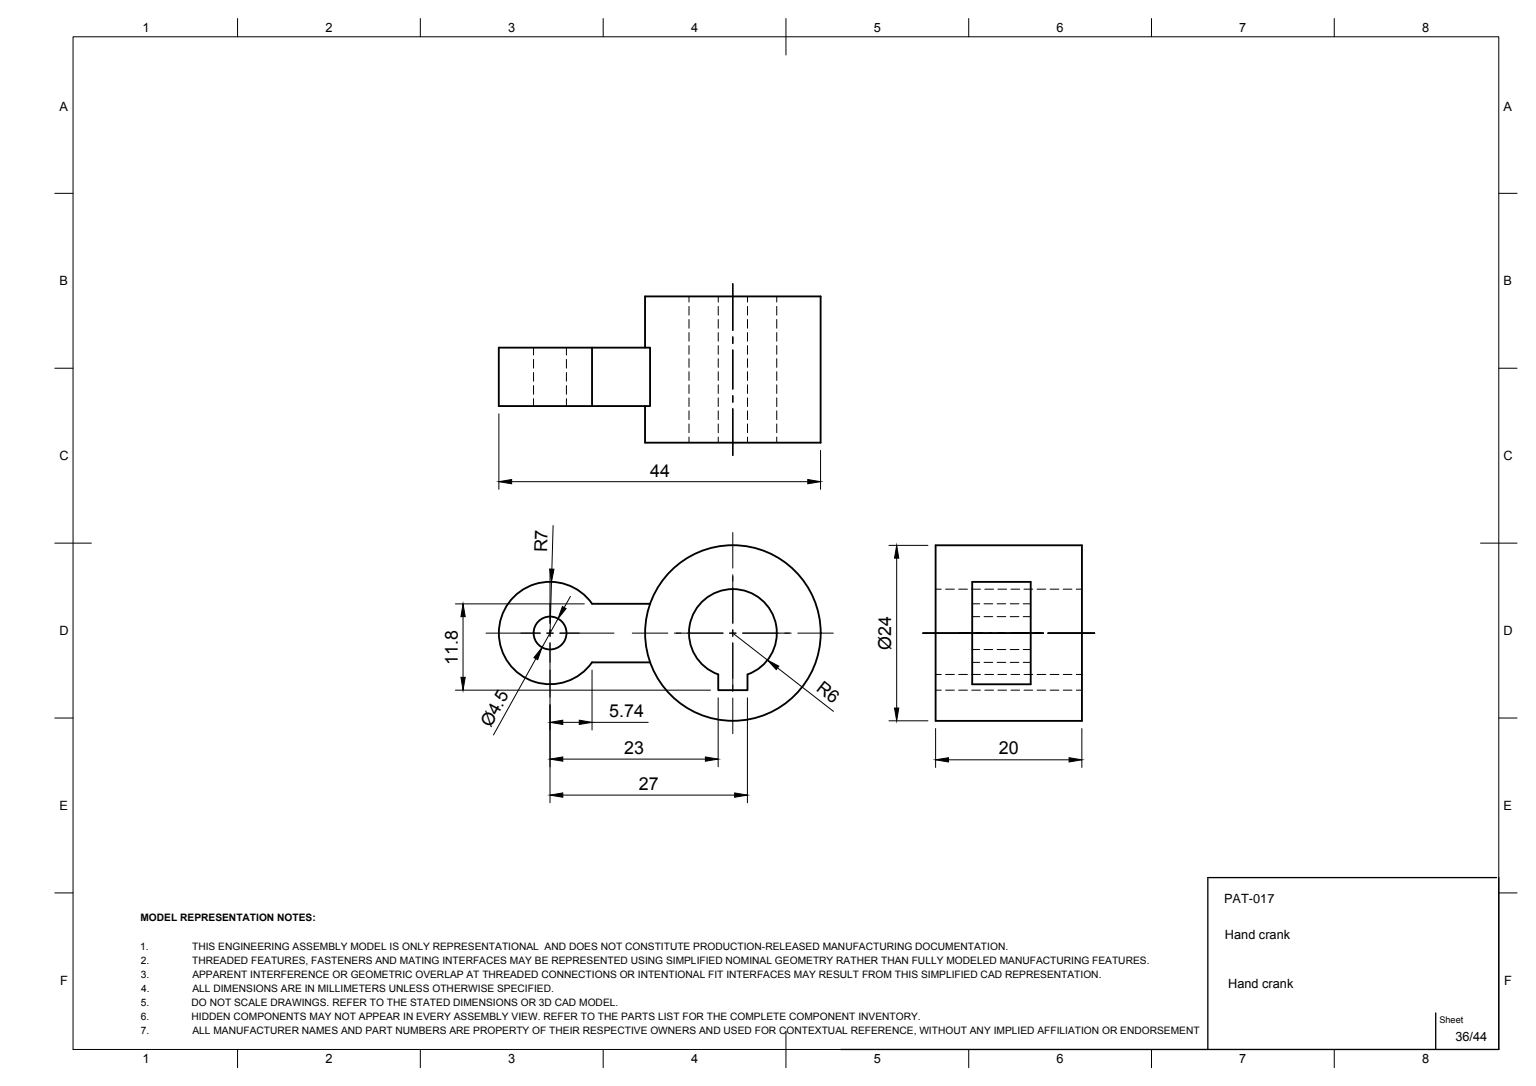
ISO-10303-21;
HEADER;
/* Generated by software containing ST-Developer
 * from STEP Tools, Inc. (www.steptools.com) 
 */

FILE_DESCRIPTION(
/* description */ ('Cam-and-follower valve demonstrator'),
/* implementation_level */ '2;1');

FILE_NAME(
/* name */ 'Hand crank.step',
/* time_stamp */ '2026-10-28T03:25:17-07:00',
/* author */ (''),
/* organization */ (''),
/* preprocessor_version */ 'ST-DEVELOPER v20.2',
/* originating_system */ 'Autodesk Translation Framework v15.17.0.0',
/* authorisation */ '');

FILE_SCHEMA (('AUTOMOTIVE_DESIGN { 1 0 10303 214 3 1 1 }'));
ENDSEC;

DATA;
#10=MECHANICAL_DESIGN_GEOMETRIC_PRESENTATION_REPRESENTATION('',(#446),#12896);
#367=SHAPE_REPRESENTATION_RELATIONSHIP('SRR','None',#13086,#403);
#403=ADVANCED_BREP_SHAPE_REPRESENTATION('',(#487),#12886);
#446=STYLED_ITEM('',(#13316),#487);
#487=MANIFOLD_SOLID_BREP('Body1',#6215);
#642=FACE_BOUND('',#1912,.T.);
#643=FACE_BOUND('',#1916,.T.);
#644=FACE_BOUND('',#1920,.T.);
#645=FACE_BOUND('',#1922,.T.);
#646=FACE_BOUND('',#1924,.T.);
#931=CIRCLE('',#7231,0.225);
#932=CIRCLE('',#7232,0.225);
#933=CIRCLE('',#7237,1.2);
#934=CIRCLE('',#7238,0.6);
#935=CIRCLE('',#7240,0.6);
#936=CIRCLE('',#7242,0.7);
#937=CIRCLE('',#7243,0.7);
#938=CIRCLE('',#7245,1.2);
#939=CIRCLE('',#7249,1.2);
#940=CIRCLE('',#7251,1.2);
#1077=CYLINDRICAL_SURFACE('',#7230,0.225);
#1078=CYLINDRICAL_SURFACE('',#7239,0.6);
#1079=CYLINDRICAL_SURFACE('',#7241,0.7);
#1080=CYLINDRICAL_SURFACE('',#7250,1.2);
#1392=FACE_OUTER_BOUND('',#1907,.T.);
#1393=FACE_OUTER_BOUND('',#1908,.T.);
#1394=FACE_OUTER_BOUND('',#1909,.T.);
#1395=FACE_OUTER_BOUND('',#1910,.T.);
#1396=FACE_OUTER_BOUND('',#1911,.T.);
#1397=FACE_OUTER_BOUND('',#1913,.T.);
#1398=FACE_OUTER_BOUND('',#1914,.T.);
#1399=FACE_OUTER_BOUND('',#1915,.T.);
#1400=FACE_OUTER_BOUND('',#1917,.T.);
#1401=FACE_OUTER_BOUND('',#1918,.T.);
#1402=FACE_OUTER_BOUND('',#1919,.T.);
#1403=FACE_OUTER_BOUND('',#1921,.T.);
#1404=FACE_OUTER_BOUND('',#1923,.T.);
#1907=EDGE_LOOP('',(#5329,#5330,#5331,#5332));
#1908=EDGE_LOOP('',(#5333,#5334,#5335,#5336));
#1909=EDGE_LOOP('',(#5337,#5338,#5339,#5340));
#1910=EDGE_LOOP('',(#5341,#5342,#5343,#5344));
#1911=EDGE_LOOP('',(#5345));
#1912=EDGE_LOOP('',(#5346,#5347,#5348,#5349));
#1913=EDGE_LOOP('',(#5350,#5351,#5352,#5353));
#1914=EDGE_LOOP('',(#5354,#5355,#5356,#5357));
#1915=EDGE_LOOP('',(#5358,#5359,#5360,#5361));
#1916=EDGE_LOOP('',(#5362));
#1917=EDGE_LOOP('',(#5363,#5364,#5365,#5366));
#1918=EDGE_LOOP('',(#5367,#5368,#5369,#5370));
#1919=EDGE_LOOP('',(#5371,#5372,#5373,#5374));
#1920=EDGE_LOOP('',(#5375));
#1921=EDGE_LOOP('',(#5376,#5377,#5378,#5379));
#1922=EDGE_LOOP('',(#5380,#5381,#5382,#5383));
#1923=EDGE_LOOP('',(#5384));
#1924=EDGE_LOOP('',(#5385,#5386,#5387,#5388));
#2325=LINE('',#12451,#2747);
#2326=LINE('',#12456,#2748);
#2327=LINE('',#12458,#2749);
#2328=LINE('',#12460,#2750);
#2329=LINE('',#12461,#2751);
#2330=LINE('',#12464,#2752);
#2331=LINE('',#12466,#2753);
#2332=LINE('',#12467,#2754);
#2333=LINE('',#12470,#2755);
#2334=LINE('',#12472,#2756);
#2335=LINE('',#12473,#2757);
#2336=LINE('',#12483,#2758);
#2337=LINE('',#12487,#2759);
#2338=LINE('',#12491,#2760);
#2339=LINE('',#12494,#2761);
#2340=LINE('',#12497,#2762);
#2341=LINE('',#12498,#2763);
#2342=LINE('',#12501,#2764);
#2343=LINE('',#12502,#2765);
#2344=LINE('',#12507,#2766);
#2747=VECTOR('',#8964,0.225);
#2748=VECTOR('',#8969,1.);
#2749=VECTOR('',#8970,1.);
#2750=VECTOR('',#8971,1.);
#2751=VECTOR('',#8972,1.);
#2752=VECTOR('',#8975,1.);
#2753=VECTOR('',#8976,1.);
#2754=VECTOR('',#8977,1.);
#2755=VECTOR('',#8980,1.);
#2756=VECTOR('',#8981,1.);
#2757=VECTOR('',#8982,1.);
#2758=VECTOR('',#8995,1.);
#2759=VECTOR('',#8998,1.);
#2760=VECTOR('',#9003,1.);
#2761=VECTOR('',#9006,1.);
#2762=VECTOR('',#9009,1.);
#2763=VECTOR('',#9010,1.);
#2764=VECTOR('',#9013,1.);
#2765=VECTOR('',#9014,1.);
#2766=VECTOR('',#9021,1.2);
#3256=VERTEX_POINT('',#12448);
#3257=VERTEX_POINT('',#12450);
#3258=VERTEX_POINT('',#12454);
#3259=VERTEX_POINT('',#12455);
#3260=VERTEX_POINT('',#12457);
#3261=VERTEX_POINT('',#12459);
#3262=VERTEX_POINT('',#12463);
#3263=VERTEX_POINT('',#12465);
#3264=VERTEX_POINT('',#12469);
#3265=VERTEX_POINT('',#12471);
#3266=VERTEX_POINT('',#12475);
#3267=VERTEX_POINT('',#12481);
#3268=VERTEX_POINT('',#12482);
#3269=VERTEX_POINT('',#12484);
#3270=VERTEX_POINT('',#12486);
#3271=VERTEX_POINT('',#12490);
#3272=VERTEX_POINT('',#12492);
#3273=VERTEX_POINT('',#12496);
#3274=VERTEX_POINT('',#12500);
#3275=VERTEX_POINT('',#12506);
#3961=EDGE_CURVE('',#3256,#3256,#931,.T.);
#3962=EDGE_CURVE('',#3256,#3257,#2325,.T.);
#3963=EDGE_CURVE('',#3257,#3257,#932,.T.);
#3964=EDGE_CURVE('',#3258,#3259,#2326,.T.);
#3965=EDGE_CURVE('',#3258,#3260,#2327,.T.);
#3966=EDGE_CURVE('',#3261,#3260,#2328,.T.);
#3967=EDGE_CURVE('',#3259,#3261,#2329,.T.);
#3968=EDGE_CURVE('',#3262,#3258,#2330,.T.);
#3969=EDGE_CURVE('',#3262,#3263,#2331,.T.);
#3970=EDGE_CURVE('',#3260,#3263,#2332,.T.);
#3971=EDGE_CURVE('',#3264,#3262,#2333,.T.);
#3972=EDGE_CURVE('',#3265,#3264,#2334,.T.);
#3973=EDGE_CURVE('',#3263,#3265,#2335,.T.);
#3974=EDGE_CURVE('',#3266,#3266,#933,.T.);
#3975=EDGE_CURVE('',#3265,#3261,#934,.T.);
#3976=EDGE_CURVE('',#3264,#3259,#935,.T.);
#3977=EDGE_CURVE('',#3267,#3268,#2336,.T.);
#3978=EDGE_CURVE('',#3269,#3267,#936,.T.);
#3979=EDGE_CURVE('',#3270,#3269,#2337,.T.);
#3980=EDGE_CURVE('',#3270,#3268,#937,.T.);
#3981=EDGE_CURVE('',#3270,#3271,#2338,.T.);
#3982=EDGE_CURVE('',#3272,#3271,#938,.T.);
#3983=EDGE_CURVE('',#3272,#3268,#2339,.T.);
#3984=EDGE_CURVE('',#3273,#3269,#2340,.T.);
#3985=EDGE_CURVE('',#3271,#3273,#2341,.T.);
#3986=EDGE_CURVE('',#3274,#3272,#2342,.T.);
#3987=EDGE_CURVE('',#3267,#3274,#2343,.T.);
#3988=EDGE_CURVE('',#3273,#3274,#939,.T.);
#3989=EDGE_CURVE('',#3266,#3275,#2344,.T.);
#3990=EDGE_CURVE('',#3275,#3275,#940,.T.);
#5329=ORIENTED_EDGE('',*,*,#3961,.F.);
#5330=ORIENTED_EDGE('',*,*,#3962,.T.);
#5331=ORIENTED_EDGE('',*,*,#3963,.F.);
#5332=ORIENTED_EDGE('',*,*,#3962,.F.);
#5333=ORIENTED_EDGE('',*,*,#3964,.F.);
#5334=ORIENTED_EDGE('',*,*,#3965,.T.);
#5335=ORIENTED_EDGE('',*,*,#3966,.F.);
#5336=ORIENTED_EDGE('',*,*,#3967,.F.);
#5337=ORIENTED_EDGE('',*,*,#3968,.F.);
#5338=ORIENTED_EDGE('',*,*,#3969,.T.);
#5339=ORIENTED_EDGE('',*,*,#3970,.F.);
#5340=ORIENTED_EDGE('',*,*,#3965,.F.);
#5341=ORIENTED_EDGE('',*,*,#3971,.F.);
#5342=ORIENTED_EDGE('',*,*,#3972,.F.);
#5343=ORIENTED_EDGE('',*,*,#3973,.F.);
#5344=ORIENTED_EDGE('',*,*,#3969,.F.);
#5345=ORIENTED_EDGE('',*,*,#3974,.T.);
#5346=ORIENTED_EDGE('',*,*,#3966,.T.);
#5347=ORIENTED_EDGE('',*,*,#3970,.T.);
#5348=ORIENTED_EDGE('',*,*,#3973,.T.);
#5349=ORIENTED_EDGE('',*,*,#3975,.T.);
#5350=ORIENTED_EDGE('',*,*,#3967,.T.);
#5351=ORIENTED_EDGE('',*,*,#3975,.F.);
#5352=ORIENTED_EDGE('',*,*,#3972,.T.);
#5353=ORIENTED_EDGE('',*,*,#3976,.T.);
#5354=ORIENTED_EDGE('',*,*,#3977,.F.);
#5355=ORIENTED_EDGE('',*,*,#3978,.F.);
#5356=ORIENTED_EDGE('',*,*,#3979,.F.);
#5357=ORIENTED_EDGE('',*,*,#3980,.T.);
#5358=ORIENTED_EDGE('',*,*,#3980,.F.);
#5359=ORIENTED_EDGE('',*,*,#3981,.T.);
#5360=ORIENTED_EDGE('',*,*,#3982,.F.);
#5361=ORIENTED_EDGE('',*,*,#3983,.T.);
#5362=ORIENTED_EDGE('',*,*,#3961,.T.);
#5363=ORIENTED_EDGE('',*,*,#3979,.T.);
#5364=ORIENTED_EDGE('',*,*,#3984,.F.);
#5365=ORIENTED_EDGE('',*,*,#3985,.F.);
#5366=ORIENTED_EDGE('',*,*,#3981,.F.);
#5367=ORIENTED_EDGE('',*,*,#3977,.T.);
#5368=ORIENTED_EDGE('',*,*,#3983,.F.);
#5369=ORIENTED_EDGE('',*,*,#3986,.F.);
#5370=ORIENTED_EDGE('',*,*,#3987,.F.);
#5371=ORIENTED_EDGE('',*,*,#3987,.T.);
#5372=ORIENTED_EDGE('',*,*,#3988,.F.);
#5373=ORIENTED_EDGE('',*,*,#3984,.T.);
#5374=ORIENTED_EDGE('',*,*,#3978,.T.);
#5375=ORIENTED_EDGE('',*,*,#3963,.T.);
#5376=ORIENTED_EDGE('',*,*,#3974,.F.);
#5377=ORIENTED_EDGE('',*,*,#3989,.T.);
#5378=ORIENTED_EDGE('',*,*,#3990,.T.);
#5379=ORIENTED_EDGE('',*,*,#3989,.F.);
#5380=ORIENTED_EDGE('',*,*,#3985,.T.);
#5381=ORIENTED_EDGE('',*,*,#3988,.T.);
#5382=ORIENTED_EDGE('',*,*,#3986,.T.);
#5383=ORIENTED_EDGE('',*,*,#3982,.T.);
#5384=ORIENTED_EDGE('',*,*,#3990,.F.);
#5385=ORIENTED_EDGE('',*,*,#3964,.T.);
#5386=ORIENTED_EDGE('',*,*,#3976,.F.);
#5387=ORIENTED_EDGE('',*,*,#3971,.T.);
#5388=ORIENTED_EDGE('',*,*,#3968,.T.);
#5762=PLANE('',#7233);
#5763=PLANE('',#7234);
#5764=PLANE('',#7235);
#5765=PLANE('',#7236);
#5766=PLANE('',#7244);
#5767=PLANE('',#7246);
#5768=PLANE('',#7247);
#5769=PLANE('',#7248);
#5770=PLANE('',#7252);
#6108=ADVANCED_FACE('',(#1392),#1077,.F.);
#6109=ADVANCED_FACE('',(#1393),#5762,.F.);
#6110=ADVANCED_FACE('',(#1394),#5763,.F.);
#6111=ADVANCED_FACE('',(#1395),#5764,.F.);
#6112=ADVANCED_FACE('',(#1396,#642),#5765,.T.);
#6113=ADVANCED_FACE('',(#1397),#1078,.F.);
#6114=ADVANCED_FACE('',(#1398),#1079,.T.);
#6115=ADVANCED_FACE('',(#1399,#643),#5766,.F.);
#6116=ADVANCED_FACE('',(#1400),#5767,.T.);
#6117=ADVANCED_FACE('',(#1401),#5768,.T.);
#6118=ADVANCED_FACE('',(#1402,#644),#5769,.T.);
#6119=ADVANCED_FACE('',(#1403,#645),#1080,.T.);
#6120=ADVANCED_FACE('',(#1404,#646),#5770,.F.);
#6215=CLOSED_SHELL('',(#6108,#6109,#6110,#6111,#6112,#6113,#6114,#6115,
#6116,#6117,#6118,#6119,#6120));
#7229=AXIS2_PLACEMENT_3D('',#12446,#8958,#8959);
#7230=AXIS2_PLACEMENT_3D('',#12447,#8960,#8961);
#7231=AXIS2_PLACEMENT_3D('',#12449,#8962,#8963);
#7232=AXIS2_PLACEMENT_3D('',#12452,#8965,#8966);
#7233=AXIS2_PLACEMENT_3D('',#12453,#8967,#8968);
#7234=AXIS2_PLACEMENT_3D('',#12462,#8973,#8974);
#7235=AXIS2_PLACEMENT_3D('',#12468,#8978,#8979);
#7236=AXIS2_PLACEMENT_3D('',#12474,#8983,#8984);
#7237=AXIS2_PLACEMENT_3D('',#12476,#8985,#8986);
#7238=AXIS2_PLACEMENT_3D('',#12477,#8987,#8988);
#7239=AXIS2_PLACEMENT_3D('',#12478,#8989,#8990);
#7240=AXIS2_PLACEMENT_3D('',#12479,#8991,#8992);
#7241=AXIS2_PLACEMENT_3D('',#12480,#8993,#8994);
#7242=AXIS2_PLACEMENT_3D('',#12485,#8996,#8997);
#7243=AXIS2_PLACEMENT_3D('',#12488,#8999,#9000);
#7244=AXIS2_PLACEMENT_3D('',#12489,#9001,#9002);
#7245=AXIS2_PLACEMENT_3D('',#12493,#9004,#9005);
#7246=AXIS2_PLACEMENT_3D('',#12495,#9007,#9008);
#7247=AXIS2_PLACEMENT_3D('',#12499,#9011,#9012);
#7248=AXIS2_PLACEMENT_3D('',#12503,#9015,#9016);
#7249=AXIS2_PLACEMENT_3D('',#12504,#9017,#9018);
#7250=AXIS2_PLACEMENT_3D('',#12505,#9019,#9020);
#7251=AXIS2_PLACEMENT_3D('',#12508,#9022,#9023);
#7252=AXIS2_PLACEMENT_3D('',#12509,#9024,#9025);
#8958=DIRECTION('axis',(0.,0.,1.));
#8959=DIRECTION('refdir',(1.,0.,0.));
#8960=DIRECTION('center_axis',(0.,1.,0.));
#8961=DIRECTION('ref_axis',(1.,0.,0.));
#8962=DIRECTION('center_axis',(0.,1.,0.));
#8963=DIRECTION('ref_axis',(1.,0.,0.));
#8964=DIRECTION('',(0.,1.,0.));
#8965=DIRECTION('center_axis',(0.,-1.,0.));
#8966=DIRECTION('ref_axis',(1.,0.,0.));
#8967=DIRECTION('center_axis',(-1.,0.,0.));
#8968=DIRECTION('ref_axis',(0.,0.,1.));
#8969=DIRECTION('',(0.,0.,1.));
#8970=DIRECTION('',(0.,1.,0.));
#8971=DIRECTION('',(0.,0.,-1.));
#8972=DIRECTION('',(0.,1.,0.));
#8973=DIRECTION('center_axis',(0.,0.,-1.));
#8974=DIRECTION('ref_axis',(-1.,0.,0.));
#8975=DIRECTION('',(-1.,0.,0.));
#8976=DIRECTION('',(0.,1.,0.));
#8977=DIRECTION('',(1.,0.,0.));
#8978=DIRECTION('center_axis',(1.,0.,0.));
#8979=DIRECTION('ref_axis',(0.,0.,-1.));
#8980=DIRECTION('',(0.,0.,-1.));
#8981=DIRECTION('',(0.,-1.,0.));
#8982=DIRECTION('',(0.,0.,1.));
#8983=DIRECTION('center_axis',(0.,1.,0.));
#8984=DIRECTION('ref_axis',(1.,0.,0.));
#8985=DIRECTION('center_axis',(0.,1.,0.));
#8986=DIRECTION('ref_axis',(1.,0.,0.));
#8987=DIRECTION('center_axis',(0.,-1.,0.));
#8988=DIRECTION('ref_axis',(1.,0.,0.));
#8989=DIRECTION('center_axis',(0.,1.,0.));
#8990=DIRECTION('ref_axis',(-1.83697019872103E-16,0.,1.));
#8991=DIRECTION('center_axis',(0.,-1.,0.));
#8992=DIRECTION('ref_axis',(1.,0.,0.));
#8993=DIRECTION('center_axis',(0.,1.,0.));
#8994=DIRECTION('ref_axis',(1.,0.,0.));
#8995=DIRECTION('',(0.,-1.,0.));
#8996=DIRECTION('center_axis',(0.,1.,0.));
#8997=DIRECTION('ref_axis',(1.,0.,0.));
#8998=DIRECTION('',(0.,1.,0.));
#8999=DIRECTION('center_axis',(0.,1.,0.));
#9000=DIRECTION('ref_axis',(1.,0.,0.));
#9001=DIRECTION('center_axis',(0.,1.,0.));
#9002=DIRECTION('ref_axis',(1.,0.,0.));
#9003=DIRECTION('',(-1.,0.,0.));
#9004=DIRECTION('center_axis',(0.,-1.,0.));
#9005=DIRECTION('ref_axis',(1.,0.,0.));
#9006=DIRECTION('',(1.,0.,0.));
#9007=DIRECTION('center_axis',(0.,0.,1.));
#9008=DIRECTION('ref_axis',(1.,0.,0.));
#9009=DIRECTION('',(1.,0.,0.));
#9010=DIRECTION('',(0.,1.,0.));
#9011=DIRECTION('center_axis',(0.,0.,-1.));
#9012=DIRECTION('ref_axis',(-1.,0.,0.));
#9013=DIRECTION('',(0.,-1.,0.));
#9014=DIRECTION('',(-1.,0.,0.));
#9015=DIRECTION('center_axis',(0.,1.,0.));
#9016=DIRECTION('ref_axis',(0.,0.,1.));
#9017=DIRECTION('center_axis',(0.,1.,0.));
#9018=DIRECTION('ref_axis',(1.,0.,0.));
#9019=DIRECTION('center_axis',(0.,1.,0.));
#9020=DIRECTION('ref_axis',(1.,0.,0.));
#9021=DIRECTION('',(0.,-1.,0.));
#9022=DIRECTION('center_axis',(0.,1.,0.));
#9023=DIRECTION('ref_axis',(1.,0.,0.));
#9024=DIRECTION('center_axis',(0.,1.,0.));
#9025=DIRECTION('ref_axis',(1.,0.,0.));
#12446=CARTESIAN_POINT('',(0.,0.,0.));
#12447=CARTESIAN_POINT('Origin',(2.5,4.9,4.));
#12448=CARTESIAN_POINT('',(2.275,5.,4.));
#12449=CARTESIAN_POINT('Origin',(2.5,5.,4.));
#12450=CARTESIAN_POINT('',(2.275,5.8,4.));
#12451=CARTESIAN_POINT('',(2.275,4.9,4.));
#12452=CARTESIAN_POINT('Origin',(2.5,5.8,4.));
#12453=CARTESIAN_POINT('Origin',(-0.2,4.4,3.22));
#12454=CARTESIAN_POINT('',(-0.2,4.5,3.22));
#12455=CARTESIAN_POINT('',(-0.2,4.5,3.43431457505076));
#12456=CARTESIAN_POINT('',(-0.2,4.5,3.61));
#12457=CARTESIAN_POINT('',(-0.2,6.5,3.22));
#12458=CARTESIAN_POINT('',(-0.2,4.4,3.22));
#12459=CARTESIAN_POINT('',(-0.2,6.5,3.43431457505076));
#12460=CARTESIAN_POINT('',(-0.2,6.5,3.61));
#12461=CARTESIAN_POINT('',(-0.2,4.5,3.43431457505076));
#12462=CARTESIAN_POINT('Origin',(0.2,4.4,3.22));
#12463=CARTESIAN_POINT('',(0.2,4.5,3.22));
#12464=CARTESIAN_POINT('',(0.1,4.5,3.22));
#12465=CARTESIAN_POINT('',(0.2,6.5,3.22));
#12466=CARTESIAN_POINT('',(0.2,4.4,3.22));
#12467=CARTESIAN_POINT('',(0.1,6.5,3.22));
#12468=CARTESIAN_POINT('Origin',(0.2,4.4,4.));
#12469=CARTESIAN_POINT('',(0.2,4.5,3.43431457505076));
#12470=CARTESIAN_POINT('',(0.2,4.5,4.));
#12471=CARTESIAN_POINT('',(0.2,6.5,3.43431457505076));
#12472=CARTESIAN_POINT('',(0.2,4.5,3.43431457505076));
#12473=CARTESIAN_POINT('',(0.2,6.5,4.));
#12474=CARTESIAN_POINT('Origin',(0.,6.5,4.));
#12475=CARTESIAN_POINT('',(-1.2,6.5,4.));
#12476=CARTESIAN_POINT('Origin',(0.,6.5,4.));
#12477=CARTESIAN_POINT('Origin',(0.,6.5,4.));
#12478=CARTESIAN_POINT('Origin',(0.,4.5,4.));
#12479=CARTESIAN_POINT('Origin',(0.,4.5,4.));
#12480=CARTESIAN_POINT('Origin',(2.5,5.,4.));
#12481=CARTESIAN_POINT('',(1.9255437353462,5.8,3.6));
#12482=CARTESIAN_POINT('',(1.9255437353462,5.,3.6));
#12483=CARTESIAN_POINT('',(1.9255437353462,5.,3.6));
#12484=CARTESIAN_POINT('',(1.9255437353462,5.8,4.4));
#12485=CARTESIAN_POINT('Origin',(2.5,5.8,4.));
#12486=CARTESIAN_POINT('',(1.9255437353462,5.,4.4));
#12487=CARTESIAN_POINT('',(1.9255437353462,5.,4.4));
#12488=CARTESIAN_POINT('Origin',(2.5,5.,4.));
#12489=CARTESIAN_POINT('Origin',(1.25,5.,4.));
#12490=CARTESIAN_POINT('',(1.13137084989848,5.,4.4));
#12491=CARTESIAN_POINT('',(2.5,5.,4.4));
#12492=CARTESIAN_POINT('',(1.13137084989848,5.,3.6));
#12493=CARTESIAN_POINT('Origin',(0.,5.,4.));
#12494=CARTESIAN_POINT('',(0.,5.,3.6));
#12495=CARTESIAN_POINT('Origin',(0.,5.,4.4));
#12496=CARTESIAN_POINT('',(1.13137084989848,5.8,4.4));
#12497=CARTESIAN_POINT('',(2.5,5.8,4.4));
#12498=CARTESIAN_POINT('',(1.13137084989848,4.5,4.4));
#12499=CARTESIAN_POINT('Origin',(2.5,5.,3.6));
#12500=CARTESIAN_POINT('',(1.13137084989848,5.8,3.6));
#12501=CARTESIAN_POINT('',(1.13137084989848,4.5,3.6));
#12502=CARTESIAN_POINT('',(0.,5.8,3.6));
#12503=CARTESIAN_POINT('Origin',(1.25,5.8,4.));
#12504=CARTESIAN_POINT('Origin',(0.,5.8,4.));
#12505=CARTESIAN_POINT('Origin',(0.,4.5,4.));
#12506=CARTESIAN_POINT('',(-1.2,4.5,4.));
#12507=CARTESIAN_POINT('',(-1.2,4.5,4.));
#12508=CARTESIAN_POINT('Origin',(0.,4.5,4.));
#12509=CARTESIAN_POINT('Origin',(0.,4.5,4.));
#12843=UNCERTAINTY_MEASURE_WITH_UNIT(LENGTH_MEASURE(0.001),#12897,
'DISTANCE_ACCURACY_VALUE',
'Maximum model space distance between geometric entities at asserted c
onnectivities');
#12853=UNCERTAINTY_MEASURE_WITH_UNIT(LENGTH_MEASURE(0.001),#12897,
'DISTANCE_ACCURACY_VALUE',
'Maximum model space distance between geometric entities at asserted c
onnectivities');
#12886=(
GEOMETRIC_REPRESENTATION_CONTEXT(3)
GLOBAL_UNCERTAINTY_ASSIGNED_CONTEXT((#12843))
GLOBAL_UNIT_ASSIGNED_CONTEXT((#12897,#12899,#12900))
REPRESENTATION_CONTEXT('','3D')
);
#12896=(
GEOMETRIC_REPRESENTATION_CONTEXT(3)
GLOBAL_UNCERTAINTY_ASSIGNED_CONTEXT((#12853))
GLOBAL_UNIT_ASSIGNED_CONTEXT((#12897,#12899,#12900))
REPRESENTATION_CONTEXT('','3D')
);
#12897=(
LENGTH_UNIT()
NAMED_UNIT(*)
SI_UNIT(.CENTI.,.METRE.)
);
#12899=(
NAMED_UNIT(*)
PLANE_ANGLE_UNIT()
SI_UNIT($,.RADIAN.)
);
#12900=(
NAMED_UNIT(*)
SI_UNIT($,.STERADIAN.)
SOLID_ANGLE_UNIT()
);
#12933=SHAPE_DEFINITION_REPRESENTATION(#12982,#13086);
#12982=PRODUCT_DEFINITION_SHAPE('',$,#13129);
#13086=SHAPE_REPRESENTATION('',(#7229),#12886);
#13096=PRODUCT_DEFINITION_CONTEXT('part definition',#13224,'design');
#13129=PRODUCT_DEFINITION('Hand crank','Hand crank',#13171,#13096);
#13171=PRODUCT_DEFINITION_FORMATION('',$,#13258);
#13224=APPLICATION_CONTEXT(
'Core Data for Automotive Mechanical Design Process');
#13225=PRODUCT_CONTEXT('part definition',#13224,'mechanical');
#13258=PRODUCT('Hand crank','Hand crank','Hand crank',(#13225));
#13310=COLOUR_RGB('Light Blue',0.38,0.62,0.78);
#13311=FILL_AREA_STYLE_COLOUR('',#13310);
#13312=FILL_AREA_STYLE('',(#13311));
#13313=SURFACE_STYLE_FILL_AREA(#13312);
#13314=SURFACE_SIDE_STYLE('',(#13313));
#13315=SURFACE_STYLE_USAGE(.BOTH.,#13314);
#13316=PRESENTATION_STYLE_ASSIGNMENT((#13315));
ENDSEC;
END-ISO-10303-21;
